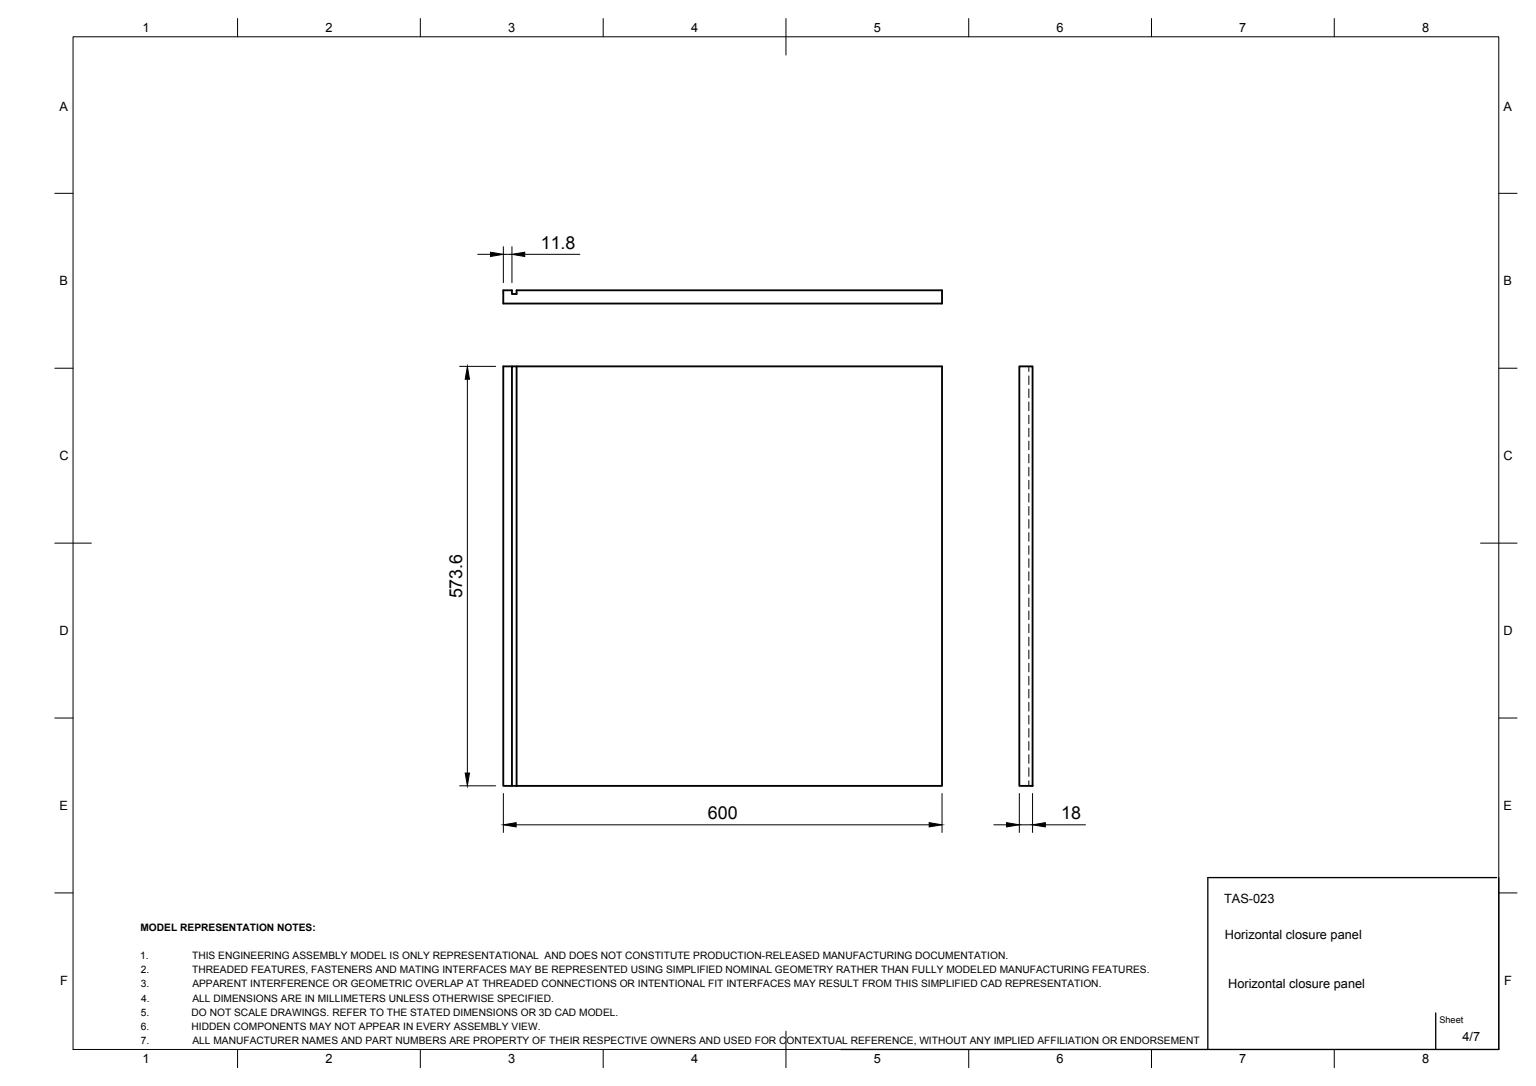
ISO-10303-21;
HEADER;
/* Generated by software containing ST-Developer
 * from STEP Tools, Inc. (www.steptools.com) 
 */

FILE_DESCRIPTION(
/* description */ (''),
/* implementation_level */ '2;1');

FILE_NAME(
/* name */ 'Horizontal closure panel.step',
/* time_stamp */ '2026-11-15T17:51:54-08:00',
/* author */ (''),
/* organization */ (''),
/* preprocessor_version */ 'ST-DEVELOPER v20.2',
/* originating_system */ 'Autodesk Translation Framework v15.17.0.0',
/* authorisation */ '');

FILE_SCHEMA (('AUTOMOTIVE_DESIGN { 1 0 10303 214 3 1 1 }'));
ENDSEC;

DATA;
#10=MECHANICAL_DESIGN_GEOMETRIC_PRESENTATION_REPRESENTATION('',(#118),#2860);
#108=SHAPE_REPRESENTATION_RELATIONSHIP('SRR','None',#2903,#113);
#113=ADVANCED_BREP_SHAPE_REPRESENTATION('',(#123),#2856);
#118=STYLED_ITEM('',(#2937),#123);
#123=MANIFOLD_SOLID_BREP('Body1',#1715);
#189=PLANE('',#1848);
#190=PLANE('',#1849);
#191=PLANE('',#1850);
#192=PLANE('',#1851);
#193=PLANE('',#1852);
#194=PLANE('',#1853);
#195=PLANE('',#1854);
#196=PLANE('',#1855);
#197=PLANE('',#1856);
#198=PLANE('',#1857);
#275=FACE_OUTER_BOUND('',#366,.T.);
#276=FACE_OUTER_BOUND('',#367,.T.);
#277=FACE_OUTER_BOUND('',#368,.T.);
#278=FACE_OUTER_BOUND('',#369,.T.);
#279=FACE_OUTER_BOUND('',#370,.T.);
#280=FACE_OUTER_BOUND('',#371,.T.);
#281=FACE_OUTER_BOUND('',#372,.T.);
#282=FACE_OUTER_BOUND('',#373,.T.);
#283=FACE_OUTER_BOUND('',#374,.T.);
#284=FACE_OUTER_BOUND('',#375,.T.);
#366=EDGE_LOOP('',(#1520,#1521,#1522,#1523));
#367=EDGE_LOOP('',(#1524,#1525,#1526,#1527));
#368=EDGE_LOOP('',(#1528,#1529,#1530,#1531));
#369=EDGE_LOOP('',(#1532,#1533,#1534,#1535,#1536,#1537,#1538,#1539));
#370=EDGE_LOOP('',(#1540,#1541,#1542,#1543));
#371=EDGE_LOOP('',(#1544,#1545,#1546,#1547));
#372=EDGE_LOOP('',(#1548,#1549,#1550,#1551));
#373=EDGE_LOOP('',(#1552,#1553,#1554,#1555,#1556,#1557,#1558,#1559));
#374=EDGE_LOOP('',(#1560,#1561,#1562,#1563));
#375=EDGE_LOOP('',(#1564,#1565,#1566,#1567));
#551=LINE('',#2713,#760);
#552=LINE('',#2715,#761);
#553=LINE('',#2717,#762);
#554=LINE('',#2718,#763);
#555=LINE('',#2722,#764);
#556=LINE('',#2724,#765);
#557=LINE('',#2726,#766);
#558=LINE('',#2727,#767);
#559=LINE('',#2729,#768);
#560=LINE('',#2730,#769);
#561=LINE('',#2733,#770);
#562=LINE('',#2735,#771);
#563=LINE('',#2737,#772);
#564=LINE('',#2739,#773);
#565=LINE('',#2740,#774);
#566=LINE('',#2743,#775);
#567=LINE('',#2744,#776);
#568=LINE('',#2747,#777);
#569=LINE('',#2749,#778);
#570=LINE('',#2750,#779);
#571=LINE('',#2753,#780);
#572=LINE('',#2754,#781);
#573=LINE('',#2756,#782);
#574=LINE('',#2757,#783);
#760=VECTOR('',#2210,1.);
#761=VECTOR('',#2211,1.);
#762=VECTOR('',#2212,1.);
#763=VECTOR('',#2213,1.);
#764=VECTOR('',#2216,1.);
#765=VECTOR('',#2217,1.);
#766=VECTOR('',#2218,1.);
#767=VECTOR('',#2219,1.);
#768=VECTOR('',#2222,1.);
#769=VECTOR('',#2223,1.);
#770=VECTOR('',#2226,1.);
#771=VECTOR('',#2227,1.);
#772=VECTOR('',#2228,1.);
#773=VECTOR('',#2229,1.);
#774=VECTOR('',#2230,1.);
#775=VECTOR('',#2233,1.);
#776=VECTOR('',#2234,1.);
#777=VECTOR('',#2237,1.);
#778=VECTOR('',#2238,1.);
#779=VECTOR('',#2239,1.);
#780=VECTOR('',#2242,1.);
#781=VECTOR('',#2243,1.);
#782=VECTOR('',#2246,1.);
#783=VECTOR('',#2247,1.);
#931=VERTEX_POINT('',#2711);
#932=VERTEX_POINT('',#2712);
#933=VERTEX_POINT('',#2714);
#934=VERTEX_POINT('',#2716);
#935=VERTEX_POINT('',#2720);
#936=VERTEX_POINT('',#2721);
#937=VERTEX_POINT('',#2723);
#938=VERTEX_POINT('',#2725);
#939=VERTEX_POINT('',#2732);
#940=VERTEX_POINT('',#2734);
#941=VERTEX_POINT('',#2736);
#942=VERTEX_POINT('',#2738);
#943=VERTEX_POINT('',#2742);
#944=VERTEX_POINT('',#2746);
#945=VERTEX_POINT('',#2748);
#946=VERTEX_POINT('',#2752);
#1133=EDGE_CURVE('',#931,#932,#551,.T.);
#1134=EDGE_CURVE('',#933,#931,#552,.T.);
#1135=EDGE_CURVE('',#934,#933,#553,.T.);
#1136=EDGE_CURVE('',#932,#934,#554,.T.);
#1137=EDGE_CURVE('',#935,#936,#555,.T.);
#1138=EDGE_CURVE('',#937,#935,#556,.T.);
#1139=EDGE_CURVE('',#938,#937,#557,.T.);
#1140=EDGE_CURVE('',#936,#938,#558,.T.);
#1141=EDGE_CURVE('',#934,#937,#559,.T.);
#1142=EDGE_CURVE('',#938,#933,#560,.T.);
#1143=EDGE_CURVE('',#939,#931,#561,.T.);
#1144=EDGE_CURVE('',#940,#939,#562,.T.);
#1145=EDGE_CURVE('',#940,#941,#563,.T.);
#1146=EDGE_CURVE('',#941,#942,#564,.T.);
#1147=EDGE_CURVE('',#936,#942,#565,.T.);
#1148=EDGE_CURVE('',#932,#943,#566,.T.);
#1149=EDGE_CURVE('',#943,#939,#567,.T.);
#1150=EDGE_CURVE('',#941,#944,#568,.T.);
#1151=EDGE_CURVE('',#944,#945,#569,.T.);
#1152=EDGE_CURVE('',#942,#945,#570,.T.);
#1153=EDGE_CURVE('',#946,#940,#571,.T.);
#1154=EDGE_CURVE('',#946,#943,#572,.T.);
#1155=EDGE_CURVE('',#945,#935,#573,.T.);
#1156=EDGE_CURVE('',#944,#946,#574,.T.);
#1520=ORIENTED_EDGE('',*,*,#1133,.F.);
#1521=ORIENTED_EDGE('',*,*,#1134,.F.);
#1522=ORIENTED_EDGE('',*,*,#1135,.F.);
#1523=ORIENTED_EDGE('',*,*,#1136,.F.);
#1524=ORIENTED_EDGE('',*,*,#1137,.F.);
#1525=ORIENTED_EDGE('',*,*,#1138,.F.);
#1526=ORIENTED_EDGE('',*,*,#1139,.F.);
#1527=ORIENTED_EDGE('',*,*,#1140,.F.);
#1528=ORIENTED_EDGE('',*,*,#1141,.F.);
#1529=ORIENTED_EDGE('',*,*,#1135,.T.);
#1530=ORIENTED_EDGE('',*,*,#1142,.F.);
#1531=ORIENTED_EDGE('',*,*,#1139,.T.);
#1532=ORIENTED_EDGE('',*,*,#1140,.T.);
#1533=ORIENTED_EDGE('',*,*,#1142,.T.);
#1534=ORIENTED_EDGE('',*,*,#1134,.T.);
#1535=ORIENTED_EDGE('',*,*,#1143,.F.);
#1536=ORIENTED_EDGE('',*,*,#1144,.F.);
#1537=ORIENTED_EDGE('',*,*,#1145,.T.);
#1538=ORIENTED_EDGE('',*,*,#1146,.T.);
#1539=ORIENTED_EDGE('',*,*,#1147,.F.);
#1540=ORIENTED_EDGE('',*,*,#1133,.T.);
#1541=ORIENTED_EDGE('',*,*,#1148,.T.);
#1542=ORIENTED_EDGE('',*,*,#1149,.T.);
#1543=ORIENTED_EDGE('',*,*,#1143,.T.);
#1544=ORIENTED_EDGE('',*,*,#1150,.T.);
#1545=ORIENTED_EDGE('',*,*,#1151,.T.);
#1546=ORIENTED_EDGE('',*,*,#1152,.F.);
#1547=ORIENTED_EDGE('',*,*,#1146,.F.);
#1548=ORIENTED_EDGE('',*,*,#1153,.T.);
#1549=ORIENTED_EDGE('',*,*,#1144,.T.);
#1550=ORIENTED_EDGE('',*,*,#1149,.F.);
#1551=ORIENTED_EDGE('',*,*,#1154,.F.);
#1552=ORIENTED_EDGE('',*,*,#1138,.T.);
#1553=ORIENTED_EDGE('',*,*,#1155,.F.);
#1554=ORIENTED_EDGE('',*,*,#1151,.F.);
#1555=ORIENTED_EDGE('',*,*,#1156,.T.);
#1556=ORIENTED_EDGE('',*,*,#1154,.T.);
#1557=ORIENTED_EDGE('',*,*,#1148,.F.);
#1558=ORIENTED_EDGE('',*,*,#1136,.T.);
#1559=ORIENTED_EDGE('',*,*,#1141,.T.);
#1560=ORIENTED_EDGE('',*,*,#1137,.T.);
#1561=ORIENTED_EDGE('',*,*,#1147,.T.);
#1562=ORIENTED_EDGE('',*,*,#1152,.T.);
#1563=ORIENTED_EDGE('',*,*,#1155,.T.);
#1564=ORIENTED_EDGE('',*,*,#1156,.F.);
#1565=ORIENTED_EDGE('',*,*,#1150,.F.);
#1566=ORIENTED_EDGE('',*,*,#1145,.F.);
#1567=ORIENTED_EDGE('',*,*,#1153,.F.);
#1689=ADVANCED_FACE('',(#275),#189,.F.);
#1690=ADVANCED_FACE('',(#276),#190,.F.);
#1691=ADVANCED_FACE('',(#277),#191,.T.);
#1692=ADVANCED_FACE('',(#278),#192,.T.);
#1693=ADVANCED_FACE('',(#279),#193,.T.);
#1694=ADVANCED_FACE('',(#280),#194,.T.);
#1695=ADVANCED_FACE('',(#281),#195,.T.);
#1696=ADVANCED_FACE('',(#282),#196,.T.);
#1697=ADVANCED_FACE('',(#283),#197,.T.);
#1698=ADVANCED_FACE('',(#284),#198,.F.);
#1715=CLOSED_SHELL('',(#1689,#1690,#1691,#1692,#1693,#1694,#1695,#1696,
#1697,#1698));
#1847=AXIS2_PLACEMENT_3D('',#2709,#2206,#2207);
#1848=AXIS2_PLACEMENT_3D('',#2710,#2208,#2209);
#1849=AXIS2_PLACEMENT_3D('',#2719,#2214,#2215);
#1850=AXIS2_PLACEMENT_3D('',#2728,#2220,#2221);
#1851=AXIS2_PLACEMENT_3D('',#2731,#2224,#2225);
#1852=AXIS2_PLACEMENT_3D('',#2741,#2231,#2232);
#1853=AXIS2_PLACEMENT_3D('',#2745,#2235,#2236);
#1854=AXIS2_PLACEMENT_3D('',#2751,#2240,#2241);
#1855=AXIS2_PLACEMENT_3D('',#2755,#2244,#2245);
#1856=AXIS2_PLACEMENT_3D('',#2758,#2248,#2249);
#1857=AXIS2_PLACEMENT_3D('',#2759,#2250,#2251);
#2206=DIRECTION('axis',(0.,0.,1.));
#2207=DIRECTION('refdir',(1.,0.,0.));
#2208=DIRECTION('center_axis',(0.,-1.,0.));
#2209=DIRECTION('ref_axis',(1.,0.,0.));
#2210=DIRECTION('',(-1.,0.,0.));
#2211=DIRECTION('',(0.,0.,1.));
#2212=DIRECTION('',(1.,0.,0.));
#2213=DIRECTION('',(0.,0.,-1.));
#2214=DIRECTION('center_axis',(0.,1.,0.));
#2215=DIRECTION('ref_axis',(-1.,0.,0.));
#2216=DIRECTION('',(1.,0.,0.));
#2217=DIRECTION('',(0.,0.,1.));
#2218=DIRECTION('',(-1.,0.,0.));
#2219=DIRECTION('',(0.,0.,-1.));
#2220=DIRECTION('center_axis',(0.,0.,1.));
#2221=DIRECTION('ref_axis',(1.,0.,0.));
#2222=DIRECTION('',(0.,1.,0.));
#2223=DIRECTION('',(0.,-1.,0.));
#2224=DIRECTION('center_axis',(1.,0.,0.));
#2225=DIRECTION('ref_axis',(0.,1.,0.));
#2226=DIRECTION('',(0.,1.,0.));
#2227=DIRECTION('',(0.,0.,1.));
#2228=DIRECTION('',(0.,1.,0.));
#2229=DIRECTION('',(0.,0.,1.));
#2230=DIRECTION('',(0.,1.,0.));
#2231=DIRECTION('center_axis',(0.,0.,1.));
#2232=DIRECTION('ref_axis',(1.,0.,0.));
#2233=DIRECTION('',(0.,-1.,0.));
#2234=DIRECTION('',(1.,0.,0.));
#2235=DIRECTION('center_axis',(0.,1.,0.));
#2236=DIRECTION('ref_axis',(-1.,0.,0.));
#2237=DIRECTION('',(-1.,0.,0.));
#2238=DIRECTION('',(0.,0.,1.));
#2239=DIRECTION('',(-1.,0.,0.));
#2240=DIRECTION('center_axis',(0.,-1.,0.));
#2241=DIRECTION('ref_axis',(1.,0.,0.));
#2242=DIRECTION('',(1.,0.,0.));
#2243=DIRECTION('',(0.,0.,1.));
#2244=DIRECTION('center_axis',(-1.,0.,0.));
#2245=DIRECTION('ref_axis',(0.,-1.,0.));
#2246=DIRECTION('',(0.,-1.,0.));
#2247=DIRECTION('',(0.,-1.,0.));
#2248=DIRECTION('center_axis',(0.,0.,1.));
#2249=DIRECTION('ref_axis',(1.,0.,0.));
#2250=DIRECTION('center_axis',(0.,0.,1.));
#2251=DIRECTION('ref_axis',(1.,0.,0.));
#2709=CARTESIAN_POINT('',(0.,0.,0.));
#2710=CARTESIAN_POINT('Origin',(0.,58.18,1.3));
#2711=CARTESIAN_POINT('',(57.36,58.18,1.8));
#2712=CARTESIAN_POINT('',(0.,58.18,1.8));
#2713=CARTESIAN_POINT('',(14.34,58.18,1.8));
#2714=CARTESIAN_POINT('',(57.36,58.18,1.3));
#2715=CARTESIAN_POINT('',(57.36,58.18,0.65));
#2716=CARTESIAN_POINT('',(0.,58.18,1.3));
#2717=CARTESIAN_POINT('',(0.,58.18,1.3));
#2718=CARTESIAN_POINT('',(0.,58.18,0.65));
#2719=CARTESIAN_POINT('Origin',(57.36,58.82,1.3));
#2720=CARTESIAN_POINT('',(0.,58.82,1.8));
#2721=CARTESIAN_POINT('',(57.36,58.82,1.8));
#2722=CARTESIAN_POINT('',(43.02,58.82,1.8));
#2723=CARTESIAN_POINT('',(0.,58.82,1.3));
#2724=CARTESIAN_POINT('',(0.,58.82,0.65));
#2725=CARTESIAN_POINT('',(57.36,58.82,1.3));
#2726=CARTESIAN_POINT('',(57.36,58.82,1.3));
#2727=CARTESIAN_POINT('',(57.36,58.82,0.65));
#2728=CARTESIAN_POINT('Origin',(28.68,58.5,1.3));
#2729=CARTESIAN_POINT('',(0.,59.25,1.3));
#2730=CARTESIAN_POINT('',(57.36,29.25,1.3));
#2731=CARTESIAN_POINT('Origin',(57.36,0.,0.));
#2732=CARTESIAN_POINT('',(57.36,0.,1.8));
#2733=CARTESIAN_POINT('',(57.36,0.,1.8));
#2734=CARTESIAN_POINT('',(57.36,0.,0.));
#2735=CARTESIAN_POINT('',(57.36,0.,0.));
#2736=CARTESIAN_POINT('',(57.36,60.,0.));
#2737=CARTESIAN_POINT('',(57.36,0.,0.));
#2738=CARTESIAN_POINT('',(57.36,60.,1.8));
#2739=CARTESIAN_POINT('',(57.36,60.,0.));
#2740=CARTESIAN_POINT('',(57.36,0.,1.8));
#2741=CARTESIAN_POINT('Origin',(28.68,30.,1.8));
#2742=CARTESIAN_POINT('',(0.,0.,1.8));
#2743=CARTESIAN_POINT('',(0.,60.,1.8));
#2744=CARTESIAN_POINT('',(0.,0.,1.8));
#2745=CARTESIAN_POINT('Origin',(57.36,60.,0.));
#2746=CARTESIAN_POINT('',(0.,60.,0.));
#2747=CARTESIAN_POINT('',(57.36,60.,0.));
#2748=CARTESIAN_POINT('',(0.,60.,1.8));
#2749=CARTESIAN_POINT('',(0.,60.,0.));
#2750=CARTESIAN_POINT('',(57.36,60.,1.8));
#2751=CARTESIAN_POINT('Origin',(0.,0.,0.));
#2752=CARTESIAN_POINT('',(0.,0.,0.));
#2753=CARTESIAN_POINT('',(0.,0.,0.));
#2754=CARTESIAN_POINT('',(0.,0.,0.));
#2755=CARTESIAN_POINT('Origin',(0.,60.,0.));
#2756=CARTESIAN_POINT('',(0.,60.,1.8));
#2757=CARTESIAN_POINT('',(0.,60.,0.));
#2758=CARTESIAN_POINT('Origin',(28.68,30.,1.8));
#2759=CARTESIAN_POINT('Origin',(28.68,30.,0.));
#2849=UNCERTAINTY_MEASURE_WITH_UNIT(LENGTH_MEASURE(0.001),#2861,
'DISTANCE_ACCURACY_VALUE',
'Maximum model space distance between geometric entities at asserted c
onnectivities');
#2853=UNCERTAINTY_MEASURE_WITH_UNIT(LENGTH_MEASURE(0.001),#2861,
'DISTANCE_ACCURACY_VALUE',
'Maximum model space distance between geometric entities at asserted c
onnectivities');
#2856=(
GEOMETRIC_REPRESENTATION_CONTEXT(3)
GLOBAL_UNCERTAINTY_ASSIGNED_CONTEXT((#2849))
GLOBAL_UNIT_ASSIGNED_CONTEXT((#2861,#2863,#2864))
REPRESENTATION_CONTEXT('','3D')
);
#2860=(
GEOMETRIC_REPRESENTATION_CONTEXT(3)
GLOBAL_UNCERTAINTY_ASSIGNED_CONTEXT((#2853))
GLOBAL_UNIT_ASSIGNED_CONTEXT((#2861,#2863,#2864))
REPRESENTATION_CONTEXT('','3D')
);
#2861=(
LENGTH_UNIT()
NAMED_UNIT(*)
SI_UNIT(.CENTI.,.METRE.)
);
#2863=(
NAMED_UNIT(*)
PLANE_ANGLE_UNIT()
SI_UNIT($,.RADIAN.)
);
#2864=(
NAMED_UNIT(*)
SI_UNIT($,.STERADIAN.)
SOLID_ANGLE_UNIT()
);
#2867=SHAPE_DEFINITION_REPRESENTATION(#2873,#2903);
#2873=PRODUCT_DEFINITION_SHAPE('',$,#2910);
#2903=SHAPE_REPRESENTATION('',(#1847),#2856);
#2907=PRODUCT_DEFINITION_CONTEXT('part definition',#2927,'design');
#2910=PRODUCT_DEFINITION('Horizontal closure panel',
'Horizontal closure panel',#2916,#2907);
#2916=PRODUCT_DEFINITION_FORMATION('',$,#2931);
#2927=APPLICATION_CONTEXT(
'Core Data for Automotive Mechanical Design Process');
#2928=PRODUCT_CONTEXT('part definition',#2927,'mechanical');
#2931=PRODUCT('Horizontal closure panel','Horizontal closure panel',$,(#2928));
#2937=PRESENTATION_STYLE_ASSIGNMENT((#2943));
#2943=SURFACE_STYLE_USAGE(.BOTH.,#2949);
#2949=SURFACE_SIDE_STYLE('',(#2955));
#2955=SURFACE_STYLE_FILL_AREA(#2961);
#2961=FILL_AREA_STYLE('Horizontal closure panel finish',(#2967));
#2967=FILL_AREA_STYLE_COLOUR('Horizontal closure panel finish',#2973);
#2973=COLOUR_RGB('Horizontal closure panel finish',0.662745098039216,0.823529411764706,
0.917647058823529);
ENDSEC;
END-ISO-10303-21;
